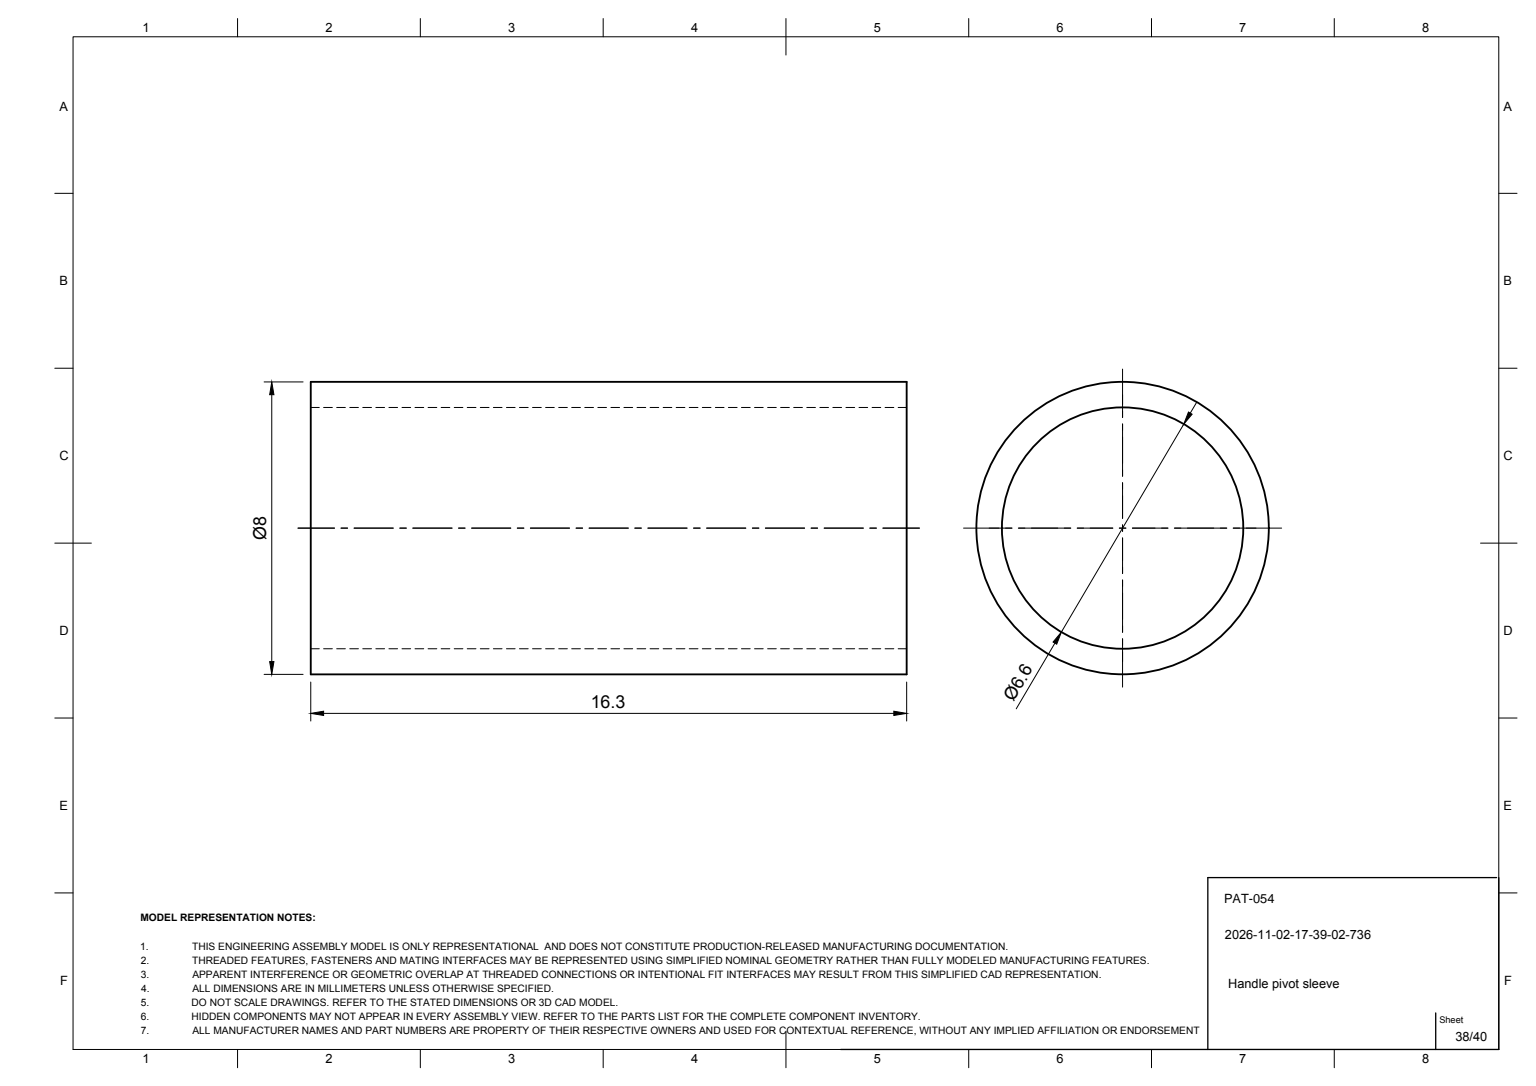
ISO-10303-21;
HEADER;
/* Generated by software containing ST-Developer
 * from STEP Tools, Inc. (www.steptools.com) 
 */

FILE_DESCRIPTION(
/* description */ ('PAT-054'),
/* implementation_level */ '2;1');

FILE_NAME(
/* name */ 'Handle pivot sleeve.step',
/* time_stamp */ '2026-10-29T16:38:13-07:00',
/* author */ (''),
/* organization */ (''),
/* preprocessor_version */ 'ST-DEVELOPER v20.2',
/* originating_system */ 'Autodesk Translation Framework v15.17.0.0',
/* authorisation */ '');

FILE_SCHEMA (('AUTOMOTIVE_DESIGN { 1 0 10303 214 3 1 1 }'));
ENDSEC;

DATA;
#10=MECHANICAL_DESIGN_GEOMETRIC_PRESENTATION_REPRESENTATION('',(#952),#33981);
#849=SHAPE_REPRESENTATION_RELATIONSHIP('SRR','None',#34227,#893);
#893=ADVANCED_BREP_SHAPE_REPRESENTATION('',(#1007),#33975);
#952=STYLED_ITEM('',(#34510),#1007);
#1007=MANIFOLD_SOLID_BREP('Body1',#13067);
#1220=FACE_BOUND('',#3181,.T.);
#1221=FACE_BOUND('',#3183,.T.);
#1539=PLANE('',#14755);
#1540=PLANE('',#14756);
#2247=FACE_OUTER_BOUND('',#3178,.T.);
#2248=FACE_OUTER_BOUND('',#3179,.T.);
#2249=FACE_OUTER_BOUND('',#3180,.T.);
#2250=FACE_OUTER_BOUND('',#3182,.T.);
#3178=EDGE_LOOP('',(#11781,#11782,#11783,#11784));
#3179=EDGE_LOOP('',(#11785,#11786,#11787,#11788));
#3180=EDGE_LOOP('',(#11789));
#3181=EDGE_LOOP('',(#11790));
#3182=EDGE_LOOP('',(#11791));
#3183=EDGE_LOOP('',(#11792));
#4096=LINE('',#33602,#5030);
#4097=LINE('',#33608,#5031);
#5030=VECTOR('',#18133,0.33);
#5031=VECTOR('',#18140,0.4);
#5546=CIRCLE('',#14750,0.33);
#5547=CIRCLE('',#14751,0.33);
#5548=CIRCLE('',#14753,0.4);
#5549=CIRCLE('',#14754,0.4);
#6680=VERTEX_POINT('',#33599);
#6681=VERTEX_POINT('',#33601);
#6682=VERTEX_POINT('',#33605);
#6683=VERTEX_POINT('',#33607);
#8390=EDGE_CURVE('',#6680,#6680,#5546,.T.);
#8391=EDGE_CURVE('',#6680,#6681,#4096,.T.);
#8392=EDGE_CURVE('',#6681,#6681,#5547,.T.);
#8393=EDGE_CURVE('',#6682,#6682,#5548,.T.);
#8394=EDGE_CURVE('',#6682,#6683,#4097,.T.);
#8395=EDGE_CURVE('',#6683,#6683,#5549,.T.);
#11781=ORIENTED_EDGE('',*,*,#8390,.F.);
#11782=ORIENTED_EDGE('',*,*,#8391,.T.);
#11783=ORIENTED_EDGE('',*,*,#8392,.T.);
#11784=ORIENTED_EDGE('',*,*,#8391,.F.);
#11785=ORIENTED_EDGE('',*,*,#8393,.F.);
#11786=ORIENTED_EDGE('',*,*,#8394,.T.);
#11787=ORIENTED_EDGE('',*,*,#8395,.T.);
#11788=ORIENTED_EDGE('',*,*,#8394,.F.);
#11789=ORIENTED_EDGE('',*,*,#8393,.T.);
#11790=ORIENTED_EDGE('',*,*,#8390,.T.);
#11791=ORIENTED_EDGE('',*,*,#8395,.F.);
#11792=ORIENTED_EDGE('',*,*,#8392,.F.);
#12278=CYLINDRICAL_SURFACE('',#14749,0.33);
#12279=CYLINDRICAL_SURFACE('',#14752,0.4);
#12959=ADVANCED_FACE('',(#2247),#12278,.F.);
#12960=ADVANCED_FACE('',(#2248),#12279,.T.);
#12961=ADVANCED_FACE('',(#2249,#1220),#1539,.T.);
#12962=ADVANCED_FACE('',(#2250,#1221),#1540,.F.);
#13067=CLOSED_SHELL('',(#12959,#12960,#12961,#12962));
#14748=AXIS2_PLACEMENT_3D('',#33597,#18127,#18128);
#14749=AXIS2_PLACEMENT_3D('',#33598,#18129,#18130);
#14750=AXIS2_PLACEMENT_3D('',#33600,#18131,#18132);
#14751=AXIS2_PLACEMENT_3D('',#33603,#18134,#18135);
#14752=AXIS2_PLACEMENT_3D('',#33604,#18136,#18137);
#14753=AXIS2_PLACEMENT_3D('',#33606,#18138,#18139);
#14754=AXIS2_PLACEMENT_3D('',#33609,#18141,#18142);
#14755=AXIS2_PLACEMENT_3D('',#33610,#18143,#18144);
#14756=AXIS2_PLACEMENT_3D('',#33611,#18145,#18146);
#18127=DIRECTION('axis',(0.,0.,1.));
#18128=DIRECTION('refdir',(1.,0.,0.));
#18129=DIRECTION('center_axis',(1.,0.,0.));
#18130=DIRECTION('ref_axis',(0.,0.,-1.));
#18131=DIRECTION('center_axis',(-1.,0.,0.));
#18132=DIRECTION('ref_axis',(0.,0.,-1.));
#18133=DIRECTION('',(-1.,0.,0.));
#18134=DIRECTION('center_axis',(-1.,0.,0.));
#18135=DIRECTION('ref_axis',(0.,0.,-1.));
#18136=DIRECTION('center_axis',(1.,0.,0.));
#18137=DIRECTION('ref_axis',(0.,0.,-1.));
#18138=DIRECTION('center_axis',(1.,0.,0.));
#18139=DIRECTION('ref_axis',(0.,0.,-1.));
#18140=DIRECTION('',(-1.,0.,0.));
#18141=DIRECTION('center_axis',(1.,0.,0.));
#18142=DIRECTION('ref_axis',(0.,0.,-1.));
#18143=DIRECTION('center_axis',(1.,0.,0.));
#18144=DIRECTION('ref_axis',(0.,0.,-1.));
#18145=DIRECTION('center_axis',(1.,0.,0.));
#18146=DIRECTION('ref_axis',(0.,0.,-1.));
#33597=CARTESIAN_POINT('',(0.,0.,0.));
#33598=CARTESIAN_POINT('Origin',(29.4,0.,6.5));
#33599=CARTESIAN_POINT('',(31.03,-4.04133443718627E-17,6.83));
#33600=CARTESIAN_POINT('Origin',(31.03,0.,6.5));
#33601=CARTESIAN_POINT('',(29.4,-4.04133443718627E-17,6.83));
#33602=CARTESIAN_POINT('',(29.4,-4.04133443718627E-17,6.83));
#33603=CARTESIAN_POINT('Origin',(29.4,0.,6.5));
#33604=CARTESIAN_POINT('Origin',(29.4,0.,6.5));
#33605=CARTESIAN_POINT('',(31.03,-4.89858719658942E-17,6.9));
#33606=CARTESIAN_POINT('Origin',(31.03,0.,6.5));
#33607=CARTESIAN_POINT('',(29.4,-4.89858719658942E-17,6.9));
#33608=CARTESIAN_POINT('',(29.4,-4.89858719658942E-17,6.9));
#33609=CARTESIAN_POINT('Origin',(29.4,0.,6.5));
#33610=CARTESIAN_POINT('Origin',(31.03,0.,6.5));
#33611=CARTESIAN_POINT('Origin',(29.4,0.,6.5));
#33923=UNCERTAINTY_MEASURE_WITH_UNIT(LENGTH_MEASURE(0.001),#33982,
'DISTANCE_ACCURACY_VALUE',
'Maximum model space distance between geometric entities at asserted c
onnectivities');
#33929=UNCERTAINTY_MEASURE_WITH_UNIT(LENGTH_MEASURE(0.001),#33982,
'DISTANCE_ACCURACY_VALUE',
'Maximum model space distance between geometric entities at asserted c
onnectivities');
#33975=(
GEOMETRIC_REPRESENTATION_CONTEXT(3)
GLOBAL_UNCERTAINTY_ASSIGNED_CONTEXT((#33923))
GLOBAL_UNIT_ASSIGNED_CONTEXT((#33982,#33984,#33985))
REPRESENTATION_CONTEXT('','3D')
);
#33981=(
GEOMETRIC_REPRESENTATION_CONTEXT(3)
GLOBAL_UNCERTAINTY_ASSIGNED_CONTEXT((#33929))
GLOBAL_UNIT_ASSIGNED_CONTEXT((#33982,#33984,#33985))
REPRESENTATION_CONTEXT('','3D')
);
#33982=(
LENGTH_UNIT()
NAMED_UNIT(*)
SI_UNIT(.CENTI.,.METRE.)
);
#33984=(
NAMED_UNIT(*)
PLANE_ANGLE_UNIT()
SI_UNIT($,.RADIAN.)
);
#33985=(
NAMED_UNIT(*)
SI_UNIT($,.STERADIAN.)
SOLID_ANGLE_UNIT()
);
#34031=SHAPE_DEFINITION_REPRESENTATION(#34115,#34227);
#34115=PRODUCT_DEFINITION_SHAPE('',$,#34279);
#34227=SHAPE_REPRESENTATION('',(#14748),#33975);
#34233=PRODUCT_DEFINITION_CONTEXT('part definition',#34388,'design');
#34279=PRODUCT_DEFINITION('Handle pivot sleeve','Handle pivot sleeve',#34330,
#34233);
#34330=PRODUCT_DEFINITION_FORMATION('',$,#34435);
#34388=APPLICATION_CONTEXT(
'Core Data for Automotive Mechanical Design Process');
#34389=PRODUCT_CONTEXT('part definition',#34388,'mechanical');
#34435=PRODUCT('Handle pivot sleeve','Handle pivot sleeve',
'Handle pivot sleeve',(#34389));
#34504=COLOUR_RGB('Sky Blue',0.24,0.69,0.87);
#34505=FILL_AREA_STYLE_COLOUR('',#34504);
#34506=FILL_AREA_STYLE('',(#34505));
#34507=SURFACE_STYLE_FILL_AREA(#34506);
#34508=SURFACE_SIDE_STYLE('',(#34507));
#34509=SURFACE_STYLE_USAGE(.BOTH.,#34508);
#34510=PRESENTATION_STYLE_ASSIGNMENT((#34509));
ENDSEC;
END-ISO-10303-21;
